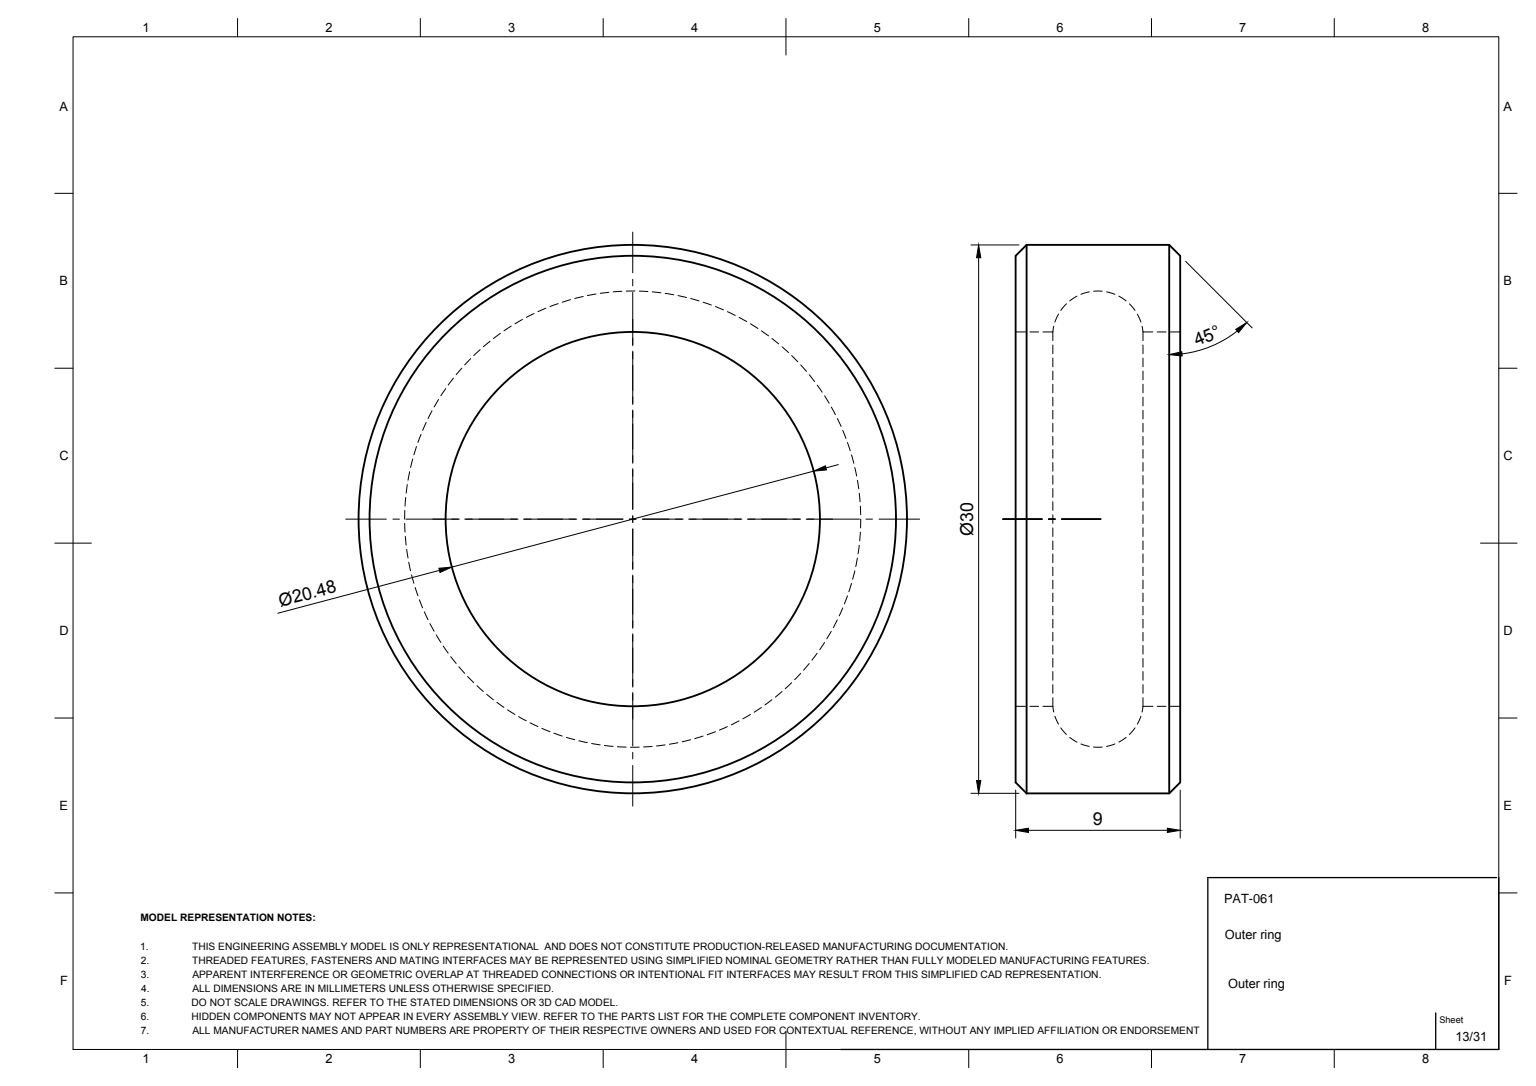
ISO-10303-21;
HEADER;
/* Generated by software containing ST-Developer
 * from STEP Tools, Inc. (www.steptools.com) 
 */

FILE_DESCRIPTION(
/* description */ ('Compact intermittent indexer'),
/* implementation_level */ '2;1');

FILE_NAME(
/* name */ 'Outer ring.step',
/* time_stamp */ '2026-10-29T16:32:17-07:00',
/* author */ (''),
/* organization */ (''),
/* preprocessor_version */ 'ST-DEVELOPER v20.2',
/* originating_system */ 'Autodesk Translation Framework v15.17.0.0',
/* authorisation */ '');

FILE_SCHEMA (('AUTOMOTIVE_DESIGN { 1 0 10303 214 3 1 1 }'));
ENDSEC;

DATA;
#10=MECHANICAL_DESIGN_GEOMETRIC_PRESENTATION_REPRESENTATION('',(#264),#10837);
#192=TOROIDAL_SURFACE('',#6210,1.,0.247676);
#201=CONICAL_SURFACE('',#6221,1.47,0.785398163397449);
#202=CONICAL_SURFACE('',#6225,1.47,0.785398163397449);
#216=SHAPE_REPRESENTATION_RELATIONSHIP('SRR','None',#10951,#240);
#240=ADVANCED_BREP_SHAPE_REPRESENTATION('',(#295),#10818);
#264=STYLED_ITEM('',(#11166),#295);
#295=MANIFOLD_SOLID_BREP('Body1',#5637);
#425=FACE_BOUND('',#1189,.T.);
#426=FACE_BOUND('',#1194,.T.);
#541=PLANE('',#6218);
#542=PLANE('',#6227);
#786=FACE_OUTER_BOUND('',#1186,.T.);
#787=FACE_OUTER_BOUND('',#1187,.T.);
#788=FACE_OUTER_BOUND('',#1188,.T.);
#789=FACE_OUTER_BOUND('',#1190,.T.);
#790=FACE_OUTER_BOUND('',#1191,.T.);
#791=FACE_OUTER_BOUND('',#1192,.T.);
#792=FACE_OUTER_BOUND('',#1193,.T.);
#793=FACE_OUTER_BOUND('',#1195,.T.);
#1186=EDGE_LOOP('',(#4260,#4261,#4262,#4263,#4264,#4265));
#1187=EDGE_LOOP('',(#4266,#4267,#4268,#4269,#4270));
#1188=EDGE_LOOP('',(#4271));
#1189=EDGE_LOOP('',(#4272));
#1190=EDGE_LOOP('',(#4273,#4274,#4275,#4276));
#1191=EDGE_LOOP('',(#4277,#4278,#4279,#4280));
#1192=EDGE_LOOP('',(#4281,#4282,#4283,#4284));
#1193=EDGE_LOOP('',(#4285));
#1194=EDGE_LOOP('',(#4286));
#1195=EDGE_LOOP('',(#4287,#4288,#4289,#4290,#4291));
#1569=LINE('',#9182,#1927);
#1570=LINE('',#9191,#1928);
#1571=LINE('',#9195,#1929);
#1572=LINE('',#9199,#1930);
#1573=LINE('',#9202,#1931);
#1927=VECTOR('',#7383,1.023815);
#1928=VECTOR('',#7394,1.47);
#1929=VECTOR('',#7399,1.5);
#1930=VECTOR('',#7404,1.47);
#1931=VECTOR('',#7409,1.023815);
#2285=CIRCLE('',#6211,1.023815);
#2286=CIRCLE('',#6212,1.023815);
#2287=CIRCLE('',#6213,0.247676);
#2288=CIRCLE('',#6214,1.023815);
#2289=CIRCLE('',#6215,1.023815);
#2290=CIRCLE('',#6217,1.023815);
#2291=CIRCLE('',#6219,1.44);
#2292=CIRCLE('',#6220,1.023815);
#2293=CIRCLE('',#6222,1.5);
#2294=CIRCLE('',#6224,1.5);
#2295=CIRCLE('',#6226,1.44);
#2664=VERTEX_POINT('',#9170);
#2665=VERTEX_POINT('',#9171);
#2666=VERTEX_POINT('',#9174);
#2667=VERTEX_POINT('',#9176);
#2668=VERTEX_POINT('',#9180);
#2669=VERTEX_POINT('',#9184);
#2670=VERTEX_POINT('',#9186);
#2671=VERTEX_POINT('',#9189);
#2672=VERTEX_POINT('',#9193);
#2673=VERTEX_POINT('',#9197);
#3252=EDGE_CURVE('',#2664,#2665,#2285,.T.);
#3253=EDGE_CURVE('',#2665,#2664,#2286,.T.);
#3254=EDGE_CURVE('',#2665,#2666,#2287,.T.);
#3255=EDGE_CURVE('',#2667,#2666,#2288,.T.);
#3256=EDGE_CURVE('',#2666,#2667,#2289,.T.);
#3257=EDGE_CURVE('',#2668,#2668,#2290,.T.);
#3258=EDGE_CURVE('',#2668,#2667,#1569,.T.);
#3259=EDGE_CURVE('',#2669,#2669,#2291,.T.);
#3260=EDGE_CURVE('',#2670,#2670,#2292,.T.);
#3261=EDGE_CURVE('',#2671,#2671,#2293,.T.);
#3262=EDGE_CURVE('',#2671,#2669,#1570,.T.);
#3263=EDGE_CURVE('',#2672,#2672,#2294,.T.);
#3264=EDGE_CURVE('',#2672,#2671,#1571,.T.);
#3265=EDGE_CURVE('',#2673,#2673,#2295,.T.);
#3266=EDGE_CURVE('',#2673,#2672,#1572,.T.);
#3267=EDGE_CURVE('',#2664,#2670,#1573,.T.);
#4260=ORIENTED_EDGE('',*,*,#3252,.F.);
#4261=ORIENTED_EDGE('',*,*,#3253,.F.);
#4262=ORIENTED_EDGE('',*,*,#3254,.T.);
#4263=ORIENTED_EDGE('',*,*,#3255,.F.);
#4264=ORIENTED_EDGE('',*,*,#3256,.F.);
#4265=ORIENTED_EDGE('',*,*,#3254,.F.);
#4266=ORIENTED_EDGE('',*,*,#3257,.T.);
#4267=ORIENTED_EDGE('',*,*,#3258,.T.);
#4268=ORIENTED_EDGE('',*,*,#3255,.T.);
#4269=ORIENTED_EDGE('',*,*,#3256,.T.);
#4270=ORIENTED_EDGE('',*,*,#3258,.F.);
#4271=ORIENTED_EDGE('',*,*,#3259,.F.);
#4272=ORIENTED_EDGE('',*,*,#3260,.T.);
#4273=ORIENTED_EDGE('',*,*,#3261,.F.);
#4274=ORIENTED_EDGE('',*,*,#3262,.T.);
#4275=ORIENTED_EDGE('',*,*,#3259,.T.);
#4276=ORIENTED_EDGE('',*,*,#3262,.F.);
#4277=ORIENTED_EDGE('',*,*,#3263,.F.);
#4278=ORIENTED_EDGE('',*,*,#3264,.T.);
#4279=ORIENTED_EDGE('',*,*,#3261,.T.);
#4280=ORIENTED_EDGE('',*,*,#3264,.F.);
#4281=ORIENTED_EDGE('',*,*,#3265,.F.);
#4282=ORIENTED_EDGE('',*,*,#3266,.T.);
#4283=ORIENTED_EDGE('',*,*,#3263,.T.);
#4284=ORIENTED_EDGE('',*,*,#3266,.F.);
#4285=ORIENTED_EDGE('',*,*,#3265,.T.);
#4286=ORIENTED_EDGE('',*,*,#3257,.F.);
#4287=ORIENTED_EDGE('',*,*,#3252,.T.);
#4288=ORIENTED_EDGE('',*,*,#3253,.T.);
#4289=ORIENTED_EDGE('',*,*,#3267,.T.);
#4290=ORIENTED_EDGE('',*,*,#3260,.F.);
#4291=ORIENTED_EDGE('',*,*,#3267,.F.);
#5229=CYLINDRICAL_SURFACE('',#6216,1.023815);
#5230=CYLINDRICAL_SURFACE('',#6223,1.5);
#5231=CYLINDRICAL_SURFACE('',#6228,1.023815);
#5429=ADVANCED_FACE('',(#786),#192,.F.);
#5430=ADVANCED_FACE('',(#787),#5229,.F.);
#5431=ADVANCED_FACE('',(#788,#425),#541,.T.);
#5432=ADVANCED_FACE('',(#789),#201,.T.);
#5433=ADVANCED_FACE('',(#790),#5230,.T.);
#5434=ADVANCED_FACE('',(#791),#202,.T.);
#5435=ADVANCED_FACE('',(#792,#426),#542,.T.);
#5436=ADVANCED_FACE('',(#793),#5231,.F.);
#5637=CLOSED_SHELL('',(#5429,#5430,#5431,#5432,#5433,#5434,#5435,#5436));
#6209=AXIS2_PLACEMENT_3D('',#9168,#7365,#7366);
#6210=AXIS2_PLACEMENT_3D('',#9169,#7367,#7368);
#6211=AXIS2_PLACEMENT_3D('',#9172,#7369,#7370);
#6212=AXIS2_PLACEMENT_3D('',#9173,#7371,#7372);
#6213=AXIS2_PLACEMENT_3D('',#9175,#7373,#7374);
#6214=AXIS2_PLACEMENT_3D('',#9177,#7375,#7376);
#6215=AXIS2_PLACEMENT_3D('',#9178,#7377,#7378);
#6216=AXIS2_PLACEMENT_3D('',#9179,#7379,#7380);
#6217=AXIS2_PLACEMENT_3D('',#9181,#7381,#7382);
#6218=AXIS2_PLACEMENT_3D('',#9183,#7384,#7385);
#6219=AXIS2_PLACEMENT_3D('',#9185,#7386,#7387);
#6220=AXIS2_PLACEMENT_3D('',#9187,#7388,#7389);
#6221=AXIS2_PLACEMENT_3D('',#9188,#7390,#7391);
#6222=AXIS2_PLACEMENT_3D('',#9190,#7392,#7393);
#6223=AXIS2_PLACEMENT_3D('',#9192,#7395,#7396);
#6224=AXIS2_PLACEMENT_3D('',#9194,#7397,#7398);
#6225=AXIS2_PLACEMENT_3D('',#9196,#7400,#7401);
#6226=AXIS2_PLACEMENT_3D('',#9198,#7402,#7403);
#6227=AXIS2_PLACEMENT_3D('',#9200,#7405,#7406);
#6228=AXIS2_PLACEMENT_3D('',#9201,#7407,#7408);
#7365=DIRECTION('axis',(0.,0.,1.));
#7366=DIRECTION('refdir',(1.,0.,0.));
#7367=DIRECTION('center_axis',(0.,-1.,0.));
#7368=DIRECTION('ref_axis',(0.,0.,-1.));
#7369=DIRECTION('center_axis',(0.,-1.,0.));
#7370=DIRECTION('ref_axis',(1.,0.,0.));
#7371=DIRECTION('center_axis',(0.,-1.,0.));
#7372=DIRECTION('ref_axis',(1.,0.,0.));
#7373=DIRECTION('center_axis',(1.,0.,1.22464679914735E-16));
#7374=DIRECTION('ref_axis',(-1.22464679914735E-16,0.,1.));
#7375=DIRECTION('center_axis',(0.,1.,0.));
#7376=DIRECTION('ref_axis',(1.,0.,0.));
#7377=DIRECTION('center_axis',(0.,1.,0.));
#7378=DIRECTION('ref_axis',(1.,0.,0.));
#7379=DIRECTION('center_axis',(0.,-1.,0.));
#7380=DIRECTION('ref_axis',(1.,0.,0.));
#7381=DIRECTION('center_axis',(0.,-1.,0.));
#7382=DIRECTION('ref_axis',(1.,0.,0.));
#7383=DIRECTION('',(0.,1.,0.));
#7384=DIRECTION('center_axis',(0.,1.,0.));
#7385=DIRECTION('ref_axis',(0.,0.,1.));
#7386=DIRECTION('center_axis',(0.,-1.,0.));
#7387=DIRECTION('ref_axis',(1.,0.,0.));
#7388=DIRECTION('center_axis',(0.,-1.,0.));
#7389=DIRECTION('ref_axis',(1.,0.,0.));
#7390=DIRECTION('center_axis',(0.,-1.,0.));
#7391=DIRECTION('ref_axis',(1.,0.,0.));
#7392=DIRECTION('center_axis',(0.,-1.,0.));
#7393=DIRECTION('ref_axis',(1.,0.,0.));
#7394=DIRECTION('',(0.707106781186548,0.707106781186547,8.65956056235494E-17));
#7395=DIRECTION('center_axis',(0.,-1.,0.));
#7396=DIRECTION('ref_axis',(1.,0.,0.));
#7397=DIRECTION('center_axis',(0.,-1.,0.));
#7398=DIRECTION('ref_axis',(1.,0.,0.));
#7399=DIRECTION('',(0.,1.,0.));
#7400=DIRECTION('center_axis',(0.,1.,0.));
#7401=DIRECTION('ref_axis',(1.,0.,0.));
#7402=DIRECTION('center_axis',(0.,-1.,0.));
#7403=DIRECTION('ref_axis',(1.,0.,0.));
#7404=DIRECTION('',(-0.707106781186548,0.707106781186547,-8.65956056235494E-17));
#7405=DIRECTION('center_axis',(0.,-1.,0.));
#7406=DIRECTION('ref_axis',(0.,0.,-1.));
#7407=DIRECTION('center_axis',(0.,-1.,0.));
#7408=DIRECTION('ref_axis',(1.,0.,0.));
#7409=DIRECTION('',(0.,1.,0.));
#9168=CARTESIAN_POINT('',(0.,0.,0.));
#9169=CARTESIAN_POINT('Origin',(0.,0.,0.));
#9170=CARTESIAN_POINT('',(-1.023815,0.246528389340863,-1.25381176266905E-16));
#9171=CARTESIAN_POINT('',(-1.25381176266905E-16,0.246528389340863,1.023815));
#9172=CARTESIAN_POINT('Origin',(0.,0.246528389340863,0.));
#9173=CARTESIAN_POINT('Origin',(0.,0.246528389340863,0.));
#9174=CARTESIAN_POINT('',(-1.25381176266905E-16,-0.246528389340863,1.023815));
#9175=CARTESIAN_POINT('Origin',(-1.22464679914735E-16,0.,1.));
#9176=CARTESIAN_POINT('',(-1.023815,-0.246528389340863,1.25381176266905E-16));
#9177=CARTESIAN_POINT('Origin',(0.,-0.246528389340863,0.));
#9178=CARTESIAN_POINT('Origin',(0.,-0.246528389340863,0.));
#9179=CARTESIAN_POINT('Origin',(0.,0.,0.));
#9180=CARTESIAN_POINT('',(-1.023815,-0.45,-1.25381176266905E-16));
#9181=CARTESIAN_POINT('Origin',(0.,-0.45,0.));
#9182=CARTESIAN_POINT('',(-1.023815,0.,-1.25381176266905E-16));
#9183=CARTESIAN_POINT('Origin',(1.44,0.45,0.));
#9184=CARTESIAN_POINT('',(-1.44,0.45,-1.76349139077219E-16));
#9185=CARTESIAN_POINT('Origin',(0.,0.45,0.));
#9186=CARTESIAN_POINT('',(-1.023815,0.45,-1.25381176266905E-16));
#9187=CARTESIAN_POINT('Origin',(0.,0.45,0.));
#9188=CARTESIAN_POINT('Origin',(0.,0.42,0.));
#9189=CARTESIAN_POINT('',(-1.5,0.39,-1.83697019872103E-16));
#9190=CARTESIAN_POINT('Origin',(0.,0.39,0.));
#9191=CARTESIAN_POINT('',(-1.47,0.42,-1.80023079474661E-16));
#9192=CARTESIAN_POINT('Origin',(0.,0.,0.));
#9193=CARTESIAN_POINT('',(-1.5,-0.39,-1.83697019872103E-16));
#9194=CARTESIAN_POINT('Origin',(0.,-0.39,0.));
#9195=CARTESIAN_POINT('',(-1.5,0.,-1.83697019872103E-16));
#9196=CARTESIAN_POINT('Origin',(0.,-0.42,0.));
#9197=CARTESIAN_POINT('',(-1.44,-0.45,-1.76349139077219E-16));
#9198=CARTESIAN_POINT('Origin',(0.,-0.45,0.));
#9199=CARTESIAN_POINT('',(-1.47,-0.42,-1.80023079474661E-16));
#9200=CARTESIAN_POINT('Origin',(1.023815,-0.45,0.));
#9201=CARTESIAN_POINT('Origin',(0.,0.,0.));
#9202=CARTESIAN_POINT('',(-1.023815,0.,-1.25381176266905E-16));
#10788=UNCERTAINTY_MEASURE_WITH_UNIT(LENGTH_MEASURE(0.001),#10838,
'DISTANCE_ACCURACY_VALUE',
'Maximum model space distance between geometric entities at asserted c
onnectivities');
#10807=UNCERTAINTY_MEASURE_WITH_UNIT(LENGTH_MEASURE(0.001),#10838,
'DISTANCE_ACCURACY_VALUE',
'Maximum model space distance between geometric entities at asserted c
onnectivities');
#10818=(
GEOMETRIC_REPRESENTATION_CONTEXT(3)
GLOBAL_UNCERTAINTY_ASSIGNED_CONTEXT((#10788))
GLOBAL_UNIT_ASSIGNED_CONTEXT((#10838,#10840,#10841))
REPRESENTATION_CONTEXT('','3D')
);
#10837=(
GEOMETRIC_REPRESENTATION_CONTEXT(3)
GLOBAL_UNCERTAINTY_ASSIGNED_CONTEXT((#10807))
GLOBAL_UNIT_ASSIGNED_CONTEXT((#10838,#10840,#10841))
REPRESENTATION_CONTEXT('','3D')
);
#10838=(
LENGTH_UNIT()
NAMED_UNIT(*)
SI_UNIT(.CENTI.,.METRE.)
);
#10840=(
NAMED_UNIT(*)
PLANE_ANGLE_UNIT()
SI_UNIT($,.RADIAN.)
);
#10841=(
NAMED_UNIT(*)
SI_UNIT($,.STERADIAN.)
SOLID_ANGLE_UNIT()
);
#10852=SHAPE_DEFINITION_REPRESENTATION(#10881,#10951);
#10881=PRODUCT_DEFINITION_SHAPE('',$,#10981);
#10951=SHAPE_REPRESENTATION('',(#6209),#10818);
#10970=PRODUCT_DEFINITION_CONTEXT('part definition',#11059,'design');
#10981=PRODUCT_DEFINITION('Outer ring','Outer ring',#11010,#10970);
#11010=PRODUCT_DEFINITION_FORMATION('',$,#11071);
#11059=APPLICATION_CONTEXT(
'Core Data for Automotive Mechanical Design Process');
#11060=PRODUCT_CONTEXT('part definition',#11059,'mechanical');
#11071=PRODUCT('Outer ring','Outer ring','Outer ring',(#11060));
#11160=COLOUR_RGB('Grey',0.48,0.52,0.57);
#11161=FILL_AREA_STYLE_COLOUR('',#11160);
#11162=FILL_AREA_STYLE('',(#11161));
#11163=SURFACE_STYLE_FILL_AREA(#11162);
#11164=SURFACE_SIDE_STYLE('',(#11163));
#11165=SURFACE_STYLE_USAGE(.BOTH.,#11164);
#11166=PRESENTATION_STYLE_ASSIGNMENT((#11165));
ENDSEC;
END-ISO-10303-21;
